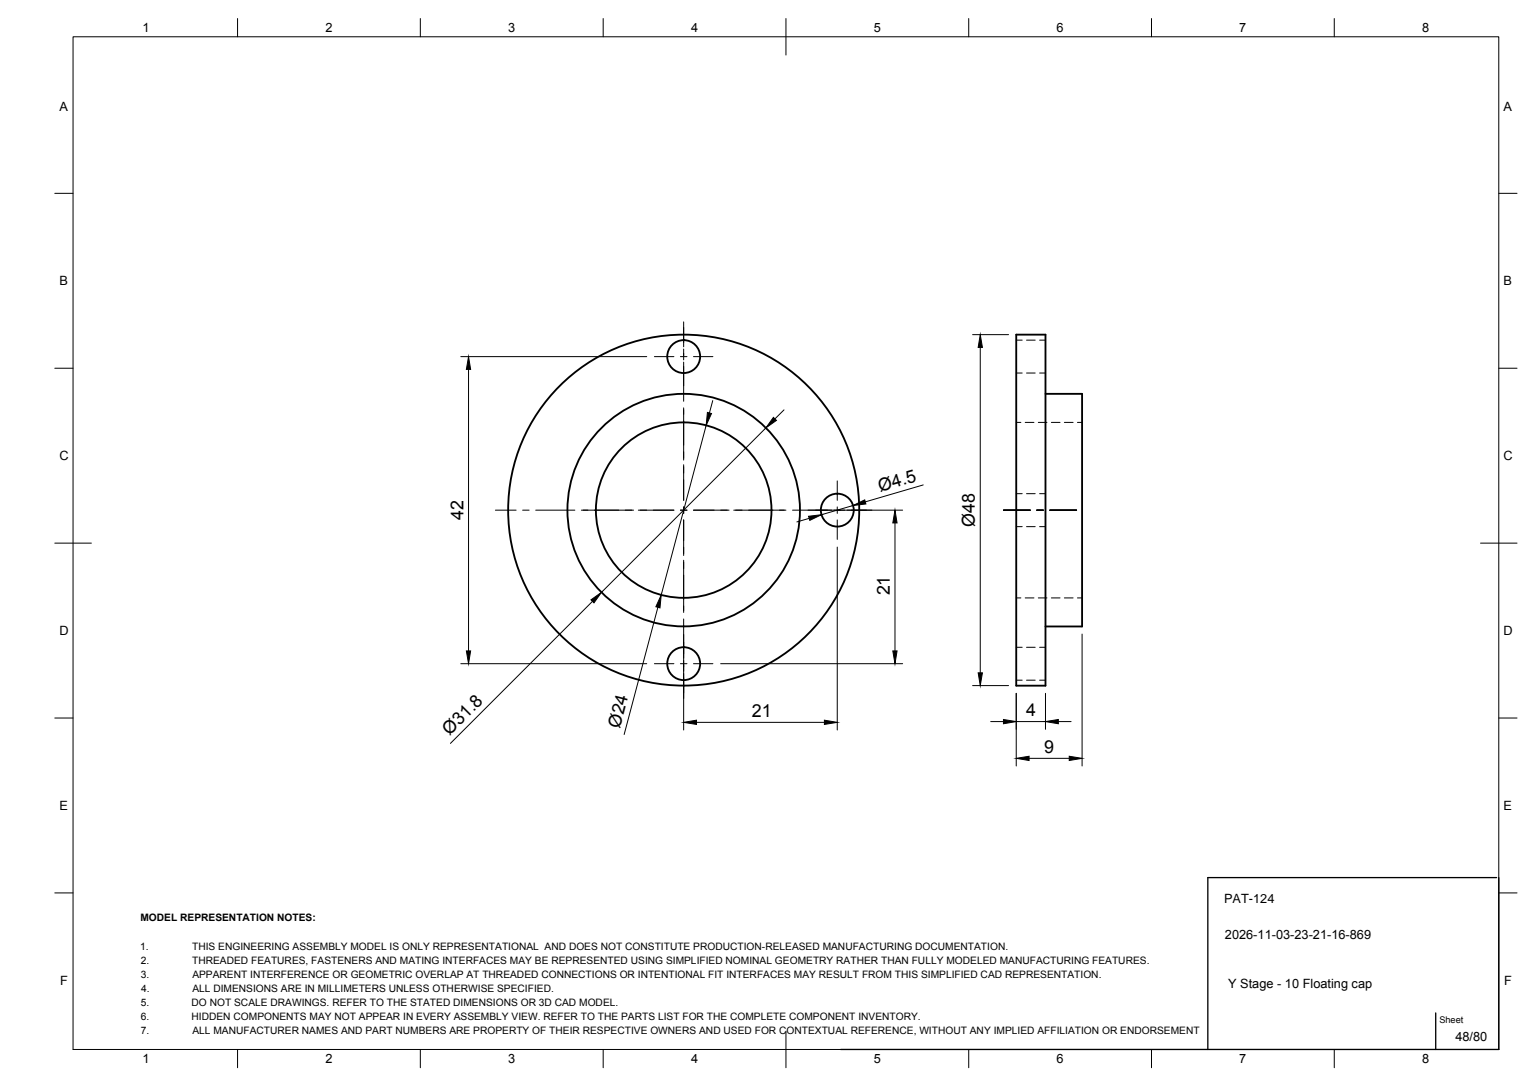
ISO-10303-21;
HEADER;
/* Generated by software containing ST-Developer
 * from STEP Tools, Inc. (www.steptools.com) 
 */

FILE_DESCRIPTION(
/* description */ ('XY cross-slide table'),
/* implementation_level */ '2;1');

FILE_NAME(
/* name */ 'Y Stage - 10 Floating cap.step',
/* time_stamp */ '2026-10-28T03:22:46-07:00',
/* author */ (''),
/* organization */ (''),
/* preprocessor_version */ 'ST-DEVELOPER v20.2',
/* originating_system */ 'Autodesk Translation Framework v15.17.0.0',
/* authorisation */ '');

FILE_SCHEMA (('AUTOMOTIVE_DESIGN { 1 0 10303 214 3 1 1 }'));
ENDSEC;

DATA;
#10=MECHANICAL_DESIGN_GEOMETRIC_PRESENTATION_REPRESENTATION('',(#1730),#62984);
#1549=SHAPE_REPRESENTATION_RELATIONSHIP('SRR','None',#63404,#1632);
#1632=ADVANCED_BREP_SHAPE_REPRESENTATION('',(#1839),#62941);
#1730=STYLED_ITEM('',(#63898),#1839);
#1839=MANIFOLD_SOLID_BREP('Body1',#23028);
#2154=FACE_BOUND('',#5182,.T.);
#2155=FACE_BOUND('',#5186,.T.);
#2156=FACE_BOUND('',#5187,.T.);
#2157=FACE_BOUND('',#5188,.T.);
#2158=FACE_BOUND('',#5189,.T.);
#2159=FACE_BOUND('',#5191,.T.);
#2160=FACE_BOUND('',#5192,.T.);
#2161=FACE_BOUND('',#5193,.T.);
#2162=FACE_BOUND('',#5194,.T.);
#2614=PLANE('',#25396);
#2615=PLANE('',#25403);
#2616=PLANE('',#25404);
#3596=FACE_OUTER_BOUND('',#5177,.T.);
#3597=FACE_OUTER_BOUND('',#5178,.T.);
#3598=FACE_OUTER_BOUND('',#5179,.T.);
#3599=FACE_OUTER_BOUND('',#5180,.T.);
#3600=FACE_OUTER_BOUND('',#5181,.T.);
#3601=FACE_OUTER_BOUND('',#5183,.T.);
#3602=FACE_OUTER_BOUND('',#5184,.T.);
#3603=FACE_OUTER_BOUND('',#5185,.T.);
#3604=FACE_OUTER_BOUND('',#5190,.T.);
#5177=EDGE_LOOP('',(#18292,#18293,#18294,#18295));
#5178=EDGE_LOOP('',(#18296,#18297,#18298,#18299));
#5179=EDGE_LOOP('',(#18300,#18301,#18302,#18303));
#5180=EDGE_LOOP('',(#18304,#18305,#18306,#18307));
#5181=EDGE_LOOP('',(#18308));
#5182=EDGE_LOOP('',(#18309));
#5183=EDGE_LOOP('',(#18310,#18311,#18312,#18313));
#5184=EDGE_LOOP('',(#18314,#18315,#18316,#18317));
#5185=EDGE_LOOP('',(#18318));
#5186=EDGE_LOOP('',(#18319));
#5187=EDGE_LOOP('',(#18320));
#5188=EDGE_LOOP('',(#18321));
#5189=EDGE_LOOP('',(#18322));
#5190=EDGE_LOOP('',(#18323));
#5191=EDGE_LOOP('',(#18324));
#5192=EDGE_LOOP('',(#18325));
#5193=EDGE_LOOP('',(#18326));
#5194=EDGE_LOOP('',(#18327));
#6731=LINE('',#48172,#8218);
#6732=LINE('',#48178,#8219);
#6733=LINE('',#48184,#8220);
#6734=LINE('',#48190,#8221);
#6735=LINE('',#48197,#8222);
#6736=LINE('',#48203,#8223);
#8218=VECTOR('',#30058,0.225);
#8219=VECTOR('',#30065,0.225);
#8220=VECTOR('',#30072,0.225);
#8221=VECTOR('',#30079,1.59);
#8222=VECTOR('',#30088,1.2);
#8223=VECTOR('',#30095,2.4);
#9405=CIRCLE('',#25385,0.225);
#9406=CIRCLE('',#25386,0.225);
#9407=CIRCLE('',#25388,0.225);
#9408=CIRCLE('',#25389,0.225);
#9409=CIRCLE('',#25391,0.225);
#9410=CIRCLE('',#25392,0.225);
#9411=CIRCLE('',#25394,1.59);
#9412=CIRCLE('',#25395,1.59);
#9413=CIRCLE('',#25397,1.2);
#9414=CIRCLE('',#25399,1.2);
#9415=CIRCLE('',#25401,2.4);
#9416=CIRCLE('',#25402,2.4);
#10909=VERTEX_POINT('',#48169);
#10910=VERTEX_POINT('',#48171);
#10911=VERTEX_POINT('',#48175);
#10912=VERTEX_POINT('',#48177);
#10913=VERTEX_POINT('',#48181);
#10914=VERTEX_POINT('',#48183);
#10915=VERTEX_POINT('',#48187);
#10916=VERTEX_POINT('',#48189);
#10917=VERTEX_POINT('',#48193);
#10918=VERTEX_POINT('',#48196);
#10919=VERTEX_POINT('',#48200);
#10920=VERTEX_POINT('',#48202);
#13530=EDGE_CURVE('',#10909,#10909,#9405,.T.);
#13531=EDGE_CURVE('',#10909,#10910,#6731,.T.);
#13532=EDGE_CURVE('',#10910,#10910,#9406,.T.);
#13533=EDGE_CURVE('',#10911,#10911,#9407,.T.);
#13534=EDGE_CURVE('',#10911,#10912,#6732,.T.);
#13535=EDGE_CURVE('',#10912,#10912,#9408,.T.);
#13536=EDGE_CURVE('',#10913,#10913,#9409,.T.);
#13537=EDGE_CURVE('',#10913,#10914,#6733,.T.);
#13538=EDGE_CURVE('',#10914,#10914,#9410,.T.);
#13539=EDGE_CURVE('',#10915,#10915,#9411,.T.);
#13540=EDGE_CURVE('',#10915,#10916,#6734,.T.);
#13541=EDGE_CURVE('',#10916,#10916,#9412,.T.);
#13542=EDGE_CURVE('',#10917,#10917,#9413,.T.);
#13543=EDGE_CURVE('',#10917,#10918,#6735,.T.);
#13544=EDGE_CURVE('',#10918,#10918,#9414,.T.);
#13545=EDGE_CURVE('',#10919,#10919,#9415,.T.);
#13546=EDGE_CURVE('',#10919,#10920,#6736,.T.);
#13547=EDGE_CURVE('',#10920,#10920,#9416,.T.);
#18292=ORIENTED_EDGE('',*,*,#13530,.F.);
#18293=ORIENTED_EDGE('',*,*,#13531,.T.);
#18294=ORIENTED_EDGE('',*,*,#13532,.F.);
#18295=ORIENTED_EDGE('',*,*,#13531,.F.);
#18296=ORIENTED_EDGE('',*,*,#13533,.F.);
#18297=ORIENTED_EDGE('',*,*,#13534,.T.);
#18298=ORIENTED_EDGE('',*,*,#13535,.F.);
#18299=ORIENTED_EDGE('',*,*,#13534,.F.);
#18300=ORIENTED_EDGE('',*,*,#13536,.F.);
#18301=ORIENTED_EDGE('',*,*,#13537,.T.);
#18302=ORIENTED_EDGE('',*,*,#13538,.F.);
#18303=ORIENTED_EDGE('',*,*,#13537,.F.);
#18304=ORIENTED_EDGE('',*,*,#13539,.F.);
#18305=ORIENTED_EDGE('',*,*,#13540,.T.);
#18306=ORIENTED_EDGE('',*,*,#13541,.F.);
#18307=ORIENTED_EDGE('',*,*,#13540,.F.);
#18308=ORIENTED_EDGE('',*,*,#13539,.T.);
#18309=ORIENTED_EDGE('',*,*,#13542,.T.);
#18310=ORIENTED_EDGE('',*,*,#13542,.F.);
#18311=ORIENTED_EDGE('',*,*,#13543,.T.);
#18312=ORIENTED_EDGE('',*,*,#13544,.T.);
#18313=ORIENTED_EDGE('',*,*,#13543,.F.);
#18314=ORIENTED_EDGE('',*,*,#13545,.F.);
#18315=ORIENTED_EDGE('',*,*,#13546,.T.);
#18316=ORIENTED_EDGE('',*,*,#13547,.T.);
#18317=ORIENTED_EDGE('',*,*,#13546,.F.);
#18318=ORIENTED_EDGE('',*,*,#13545,.T.);
#18319=ORIENTED_EDGE('',*,*,#13532,.T.);
#18320=ORIENTED_EDGE('',*,*,#13535,.T.);
#18321=ORIENTED_EDGE('',*,*,#13538,.T.);
#18322=ORIENTED_EDGE('',*,*,#13541,.T.);
#18323=ORIENTED_EDGE('',*,*,#13547,.F.);
#18324=ORIENTED_EDGE('',*,*,#13530,.T.);
#18325=ORIENTED_EDGE('',*,*,#13533,.T.);
#18326=ORIENTED_EDGE('',*,*,#13536,.T.);
#18327=ORIENTED_EDGE('',*,*,#13544,.F.);
#21385=CYLINDRICAL_SURFACE('',#25384,0.225);
#21386=CYLINDRICAL_SURFACE('',#25387,0.225);
#21387=CYLINDRICAL_SURFACE('',#25390,0.225);
#21388=CYLINDRICAL_SURFACE('',#25393,1.59);
#21389=CYLINDRICAL_SURFACE('',#25398,1.2);
#21390=CYLINDRICAL_SURFACE('',#25400,2.4);
#22377=ADVANCED_FACE('',(#3596),#21385,.F.);
#22378=ADVANCED_FACE('',(#3597),#21386,.F.);
#22379=ADVANCED_FACE('',(#3598),#21387,.F.);
#22380=ADVANCED_FACE('',(#3599),#21388,.T.);
#22381=ADVANCED_FACE('',(#3600,#2154),#2614,.T.);
#22382=ADVANCED_FACE('',(#3601),#21389,.F.);
#22383=ADVANCED_FACE('',(#3602),#21390,.T.);
#22384=ADVANCED_FACE('',(#3603,#2155,#2156,#2157,#2158),#2615,.T.);
#22385=ADVANCED_FACE('',(#3604,#2159,#2160,#2161,#2162),#2616,.F.);
#23028=CLOSED_SHELL('',(#22377,#22378,#22379,#22380,#22381,#22382,#22383,
#22384,#22385));
#25383=AXIS2_PLACEMENT_3D('',#48167,#30052,#30053);
#25384=AXIS2_PLACEMENT_3D('',#48168,#30054,#30055);
#25385=AXIS2_PLACEMENT_3D('',#48170,#30056,#30057);
#25386=AXIS2_PLACEMENT_3D('',#48173,#30059,#30060);
#25387=AXIS2_PLACEMENT_3D('',#48174,#30061,#30062);
#25388=AXIS2_PLACEMENT_3D('',#48176,#30063,#30064);
#25389=AXIS2_PLACEMENT_3D('',#48179,#30066,#30067);
#25390=AXIS2_PLACEMENT_3D('',#48180,#30068,#30069);
#25391=AXIS2_PLACEMENT_3D('',#48182,#30070,#30071);
#25392=AXIS2_PLACEMENT_3D('',#48185,#30073,#30074);
#25393=AXIS2_PLACEMENT_3D('',#48186,#30075,#30076);
#25394=AXIS2_PLACEMENT_3D('',#48188,#30077,#30078);
#25395=AXIS2_PLACEMENT_3D('',#48191,#30080,#30081);
#25396=AXIS2_PLACEMENT_3D('',#48192,#30082,#30083);
#25397=AXIS2_PLACEMENT_3D('',#48194,#30084,#30085);
#25398=AXIS2_PLACEMENT_3D('',#48195,#30086,#30087);
#25399=AXIS2_PLACEMENT_3D('',#48198,#30089,#30090);
#25400=AXIS2_PLACEMENT_3D('',#48199,#30091,#30092);
#25401=AXIS2_PLACEMENT_3D('',#48201,#30093,#30094);
#25402=AXIS2_PLACEMENT_3D('',#48204,#30096,#30097);
#25403=AXIS2_PLACEMENT_3D('',#48205,#30098,#30099);
#25404=AXIS2_PLACEMENT_3D('',#48206,#30100,#30101);
#30052=DIRECTION('axis',(0.,0.,1.));
#30053=DIRECTION('refdir',(1.,0.,0.));
#30054=DIRECTION('center_axis',(1.,0.,0.));
#30055=DIRECTION('ref_axis',(0.,0.,-1.));
#30056=DIRECTION('center_axis',(1.,0.,0.));
#30057=DIRECTION('ref_axis',(0.,0.,-1.));
#30058=DIRECTION('',(1.,0.,0.));
#30059=DIRECTION('center_axis',(-1.,0.,0.));
#30060=DIRECTION('ref_axis',(0.,0.,-1.));
#30061=DIRECTION('center_axis',(1.,0.,0.));
#30062=DIRECTION('ref_axis',(0.,0.,-1.));
#30063=DIRECTION('center_axis',(1.,0.,0.));
#30064=DIRECTION('ref_axis',(0.,0.,-1.));
#30065=DIRECTION('',(1.,0.,0.));
#30066=DIRECTION('center_axis',(-1.,0.,0.));
#30067=DIRECTION('ref_axis',(0.,0.,-1.));
#30068=DIRECTION('center_axis',(1.,0.,0.));
#30069=DIRECTION('ref_axis',(0.,0.,-1.));
#30070=DIRECTION('center_axis',(1.,0.,0.));
#30071=DIRECTION('ref_axis',(0.,0.,-1.));
#30072=DIRECTION('',(1.,0.,0.));
#30073=DIRECTION('center_axis',(-1.,0.,0.));
#30074=DIRECTION('ref_axis',(0.,0.,-1.));
#30075=DIRECTION('center_axis',(1.,0.,0.));
#30076=DIRECTION('ref_axis',(0.,0.,-1.));
#30077=DIRECTION('center_axis',(1.,0.,0.));
#30078=DIRECTION('ref_axis',(0.,0.,-1.));
#30079=DIRECTION('',(-1.,0.,0.));
#30080=DIRECTION('center_axis',(-1.,0.,0.));
#30081=DIRECTION('ref_axis',(0.,0.,-1.));
#30082=DIRECTION('center_axis',(1.,0.,0.));
#30083=DIRECTION('ref_axis',(0.,0.,-1.));
#30084=DIRECTION('center_axis',(-1.,0.,0.));
#30085=DIRECTION('ref_axis',(0.,0.,-1.));
#30086=DIRECTION('center_axis',(1.,0.,0.));
#30087=DIRECTION('ref_axis',(0.,0.,-1.));
#30088=DIRECTION('',(-1.,0.,0.));
#30089=DIRECTION('center_axis',(-1.,0.,0.));
#30090=DIRECTION('ref_axis',(0.,0.,-1.));
#30091=DIRECTION('center_axis',(1.,0.,0.));
#30092=DIRECTION('ref_axis',(0.,0.,-1.));
#30093=DIRECTION('center_axis',(1.,0.,0.));
#30094=DIRECTION('ref_axis',(0.,0.,-1.));
#30095=DIRECTION('',(-1.,0.,0.));
#30096=DIRECTION('center_axis',(1.,0.,0.));
#30097=DIRECTION('ref_axis',(0.,0.,-1.));
#30098=DIRECTION('center_axis',(1.,0.,0.));
#30099=DIRECTION('ref_axis',(0.,0.,-1.));
#30100=DIRECTION('center_axis',(1.,0.,0.));
#30101=DIRECTION('ref_axis',(0.,0.,-1.));
#48167=CARTESIAN_POINT('',(0.,0.,0.));
#48168=CARTESIAN_POINT('Origin',(1.5,-2.1,4.));
#48169=CARTESIAN_POINT('',(1.6,-2.1,4.225));
#48170=CARTESIAN_POINT('Origin',(1.6,-2.1,4.));
#48171=CARTESIAN_POINT('',(2.,-2.1,4.225));
#48172=CARTESIAN_POINT('',(1.5,-2.1,4.225));
#48173=CARTESIAN_POINT('Origin',(2.,-2.1,4.));
#48174=CARTESIAN_POINT('Origin',(1.5,2.1,4.));
#48175=CARTESIAN_POINT('',(1.6,2.1,4.225));
#48176=CARTESIAN_POINT('Origin',(1.6,2.1,4.));
#48177=CARTESIAN_POINT('',(2.,2.1,4.225));
#48178=CARTESIAN_POINT('',(1.5,2.1,4.225));
#48179=CARTESIAN_POINT('Origin',(2.,2.1,4.));
#48180=CARTESIAN_POINT('Origin',(1.5,0.,6.1));
#48181=CARTESIAN_POINT('',(1.6,-2.75545529808154E-17,6.325));
#48182=CARTESIAN_POINT('Origin',(1.6,0.,6.1));
#48183=CARTESIAN_POINT('',(2.,2.75545529808154E-17,6.325));
#48184=CARTESIAN_POINT('',(1.5,-2.75545529808154E-17,6.325));
#48185=CARTESIAN_POINT('Origin',(2.,0.,6.1));
#48186=CARTESIAN_POINT('Origin',(2.,0.,4.));
#48187=CARTESIAN_POINT('',(2.5,-1.94718841064429E-16,5.59));
#48188=CARTESIAN_POINT('Origin',(2.5,0.,4.));
#48189=CARTESIAN_POINT('',(2.,-1.94718841064429E-16,5.59));
#48190=CARTESIAN_POINT('',(2.,-1.94718841064429E-16,5.59));
#48191=CARTESIAN_POINT('Origin',(2.,0.,4.));
#48192=CARTESIAN_POINT('Origin',(2.5,0.,4.));
#48193=CARTESIAN_POINT('',(2.5,-1.46957615897682E-16,5.2));
#48194=CARTESIAN_POINT('Origin',(2.5,0.,4.));
#48195=CARTESIAN_POINT('Origin',(1.6,0.,4.));
#48196=CARTESIAN_POINT('',(1.6,-1.46957615897682E-16,5.2));
#48197=CARTESIAN_POINT('',(1.6,-1.46957615897682E-16,5.2));
#48198=CARTESIAN_POINT('Origin',(1.6,0.,4.));
#48199=CARTESIAN_POINT('Origin',(1.6,0.,4.));
#48200=CARTESIAN_POINT('',(2.,-2.93915231795365E-16,6.4));
#48201=CARTESIAN_POINT('Origin',(2.,0.,4.));
#48202=CARTESIAN_POINT('',(1.6,-2.93915231795365E-16,6.4));
#48203=CARTESIAN_POINT('',(1.6,-2.93915231795365E-16,6.4));
#48204=CARTESIAN_POINT('Origin',(1.6,0.,4.));
#48205=CARTESIAN_POINT('Origin',(2.,0.,4.));
#48206=CARTESIAN_POINT('Origin',(1.6,0.,4.));
#62842=UNCERTAINTY_MEASURE_WITH_UNIT(LENGTH_MEASURE(0.001),#62985,
'DISTANCE_ACCURACY_VALUE',
'Maximum model space distance between geometric entities at asserted c
onnectivities');
#62885=UNCERTAINTY_MEASURE_WITH_UNIT(LENGTH_MEASURE(0.001),#62985,
'DISTANCE_ACCURACY_VALUE',
'Maximum model space distance between geometric entities at asserted c
onnectivities');
#62941=(
GEOMETRIC_REPRESENTATION_CONTEXT(3)
GLOBAL_UNCERTAINTY_ASSIGNED_CONTEXT((#62842))
GLOBAL_UNIT_ASSIGNED_CONTEXT((#62985,#62987,#62988))
REPRESENTATION_CONTEXT('','3D')
);
#62984=(
GEOMETRIC_REPRESENTATION_CONTEXT(3)
GLOBAL_UNCERTAINTY_ASSIGNED_CONTEXT((#62885))
GLOBAL_UNIT_ASSIGNED_CONTEXT((#62985,#62987,#62988))
REPRESENTATION_CONTEXT('','3D')
);
#62985=(
LENGTH_UNIT()
NAMED_UNIT(*)
SI_UNIT(.CENTI.,.METRE.)
);
#62987=(
NAMED_UNIT(*)
PLANE_ANGLE_UNIT()
SI_UNIT($,.RADIAN.)
);
#62988=(
NAMED_UNIT(*)
SI_UNIT($,.STERADIAN.)
SOLID_ANGLE_UNIT()
);
#63044=SHAPE_DEFINITION_REPRESENTATION(#63222,#63404);
#63222=PRODUCT_DEFINITION_SHAPE('',$,#63503);
#63404=SHAPE_REPRESENTATION('',(#25383),#62941);
#63447=PRODUCT_DEFINITION_CONTEXT('part definition',#63743,'design');
#63503=PRODUCT_DEFINITION('Y Stage - 10 Floating cap',
'Y Stage - 10 Floating cap',#63601,#63447);
#63601=PRODUCT_DEFINITION_FORMATION('',$,#63800);
#63743=APPLICATION_CONTEXT(
'Core Data for Automotive Mechanical Design Process');
#63744=PRODUCT_CONTEXT('part definition',#63743,'mechanical');
#63800=PRODUCT('Y Stage - 10 Floating cap','Y Stage - 10 Floating cap',
'Y Stage - 10 Floating cap',(#63744));
#63892=COLOUR_RGB('Light Blue',0.38,0.62,0.78);
#63893=FILL_AREA_STYLE_COLOUR('',#63892);
#63894=FILL_AREA_STYLE('',(#63893));
#63895=SURFACE_STYLE_FILL_AREA(#63894);
#63896=SURFACE_SIDE_STYLE('',(#63895));
#63897=SURFACE_STYLE_USAGE(.BOTH.,#63896);
#63898=PRESENTATION_STYLE_ASSIGNMENT((#63897));
ENDSEC;
END-ISO-10303-21;
